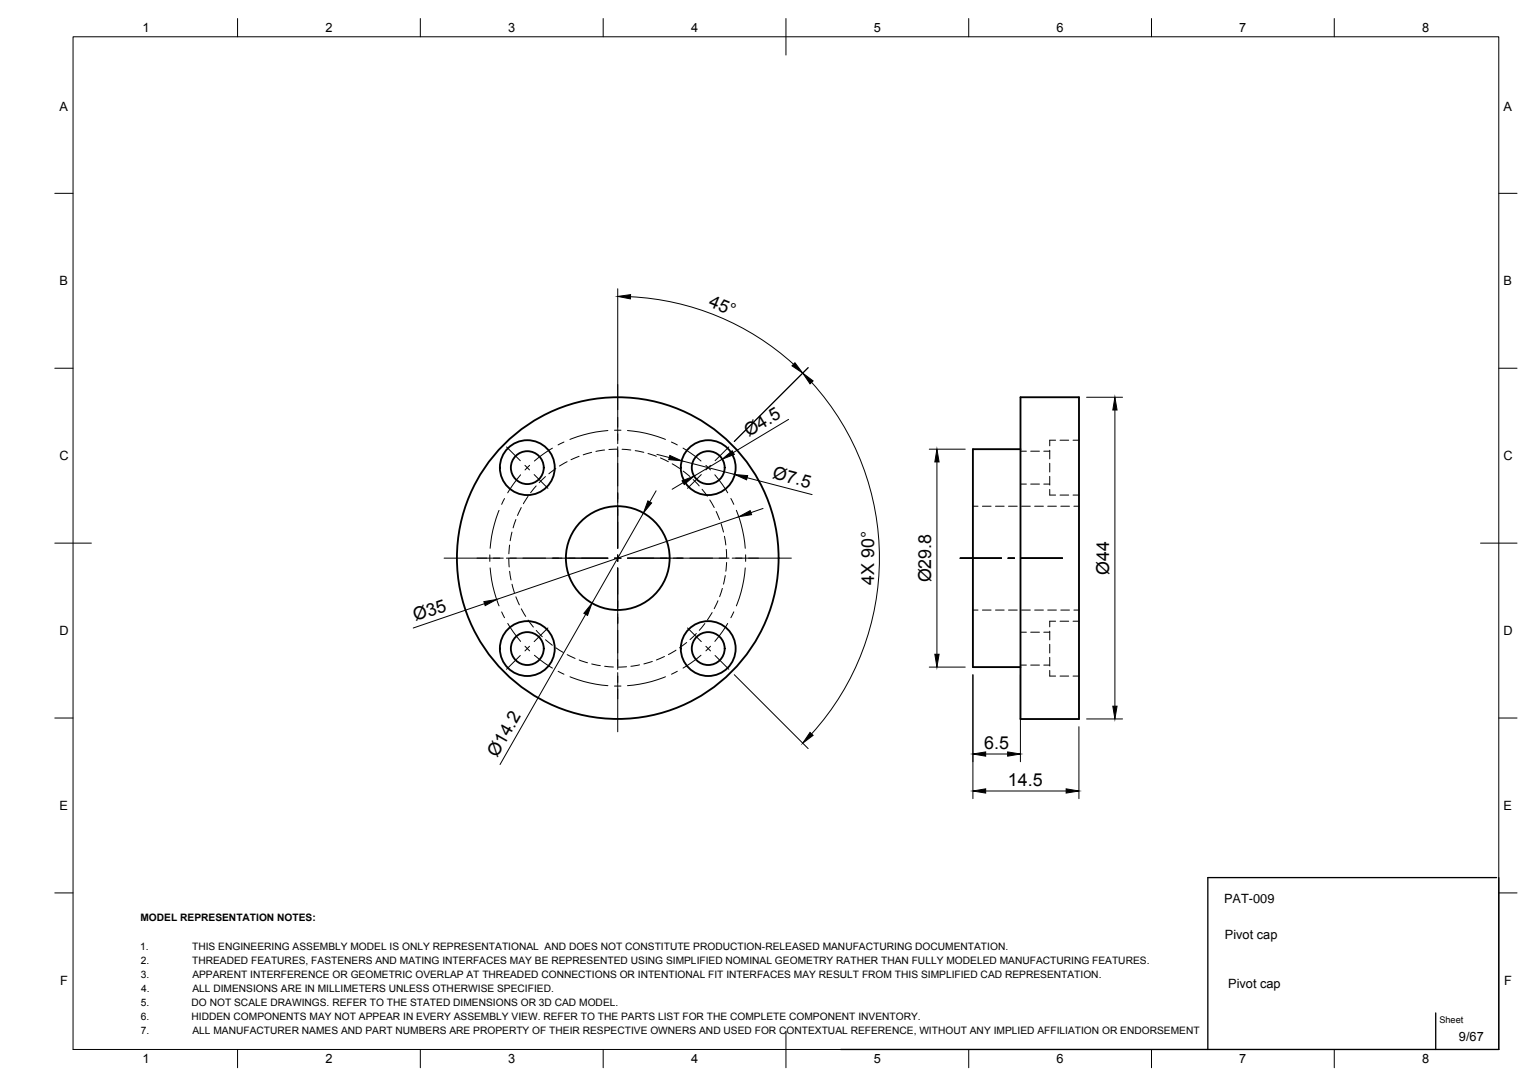
ISO-10303-21;
HEADER;
/* Generated by software containing ST-Developer
 * from STEP Tools, Inc. (www.steptools.com) 
 */

FILE_DESCRIPTION(
/* description */ ('Bell-crank linkage with push rods'),
/* implementation_level */ '2;1');

FILE_NAME(
/* name */ 'Pivot cap.step',
/* time_stamp */ '2026-10-28T03:25:15-07:00',
/* author */ (''),
/* organization */ (''),
/* preprocessor_version */ 'ST-DEVELOPER v20.2',
/* originating_system */ 'Autodesk Translation Framework v15.17.0.0',
/* authorisation */ '');

FILE_SCHEMA (('AUTOMOTIVE_DESIGN { 1 0 10303 214 3 1 1 }'));
ENDSEC;

DATA;
#10=MECHANICAL_DESIGN_GEOMETRIC_PRESENTATION_REPRESENTATION('',(#608),#16678);
#500=SHAPE_REPRESENTATION_RELATIONSHIP('SRR','None',#16916,#554);
#554=ADVANCED_BREP_SHAPE_REPRESENTATION('',(#670),#16621);
#608=STYLED_ITEM('',(#17277),#670);
#670=MANIFOLD_SOLID_BREP('Body1',#8798);
#767=FACE_BOUND('',#1872,.T.);
#768=FACE_BOUND('',#1875,.T.);
#769=FACE_BOUND('',#1878,.T.);
#770=FACE_BOUND('',#1881,.T.);
#771=FACE_BOUND('',#1888,.T.);
#772=FACE_BOUND('',#1892,.T.);
#773=FACE_BOUND('',#1893,.T.);
#774=FACE_BOUND('',#1894,.T.);
#775=FACE_BOUND('',#1895,.T.);
#776=FACE_BOUND('',#1896,.T.);
#777=FACE_BOUND('',#1898,.T.);
#778=FACE_BOUND('',#1899,.T.);
#779=FACE_BOUND('',#1900,.T.);
#780=FACE_BOUND('',#1901,.T.);
#781=FACE_BOUND('',#1902,.T.);
#996=PLANE('',#9587);
#997=PLANE('',#9592);
#998=PLANE('',#9597);
#999=PLANE('',#9602);
#1000=PLANE('',#9615);
#1001=PLANE('',#9622);
#1002=PLANE('',#9623);
#1306=FACE_OUTER_BOUND('',#1870,.T.);
#1307=FACE_OUTER_BOUND('',#1871,.T.);
#1308=FACE_OUTER_BOUND('',#1873,.T.);
#1309=FACE_OUTER_BOUND('',#1874,.T.);
#1310=FACE_OUTER_BOUND('',#1876,.T.);
#1311=FACE_OUTER_BOUND('',#1877,.T.);
#1312=FACE_OUTER_BOUND('',#1879,.T.);
#1313=FACE_OUTER_BOUND('',#1880,.T.);
#1314=FACE_OUTER_BOUND('',#1882,.T.);
#1315=FACE_OUTER_BOUND('',#1883,.T.);
#1316=FACE_OUTER_BOUND('',#1884,.T.);
#1317=FACE_OUTER_BOUND('',#1885,.T.);
#1318=FACE_OUTER_BOUND('',#1886,.T.);
#1319=FACE_OUTER_BOUND('',#1887,.T.);
#1320=FACE_OUTER_BOUND('',#1889,.T.);
#1321=FACE_OUTER_BOUND('',#1890,.T.);
#1322=FACE_OUTER_BOUND('',#1891,.T.);
#1323=FACE_OUTER_BOUND('',#1897,.T.);
#1870=EDGE_LOOP('',(#6185,#6186,#6187,#6188));
#1871=EDGE_LOOP('',(#6189));
#1872=EDGE_LOOP('',(#6190));
#1873=EDGE_LOOP('',(#6191,#6192,#6193,#6194));
#1874=EDGE_LOOP('',(#6195));
#1875=EDGE_LOOP('',(#6196));
#1876=EDGE_LOOP('',(#6197,#6198,#6199,#6200));
#1877=EDGE_LOOP('',(#6201));
#1878=EDGE_LOOP('',(#6202));
#1879=EDGE_LOOP('',(#6203,#6204,#6205,#6206));
#1880=EDGE_LOOP('',(#6207));
#1881=EDGE_LOOP('',(#6208));
#1882=EDGE_LOOP('',(#6209,#6210,#6211,#6212));
#1883=EDGE_LOOP('',(#6213,#6214,#6215,#6216));
#1884=EDGE_LOOP('',(#6217,#6218,#6219,#6220));
#1885=EDGE_LOOP('',(#6221,#6222,#6223,#6224));
#1886=EDGE_LOOP('',(#6225,#6226,#6227,#6228));
#1887=EDGE_LOOP('',(#6229));
#1888=EDGE_LOOP('',(#6230));
#1889=EDGE_LOOP('',(#6231,#6232,#6233,#6234));
#1890=EDGE_LOOP('',(#6235,#6236,#6237,#6238));
#1891=EDGE_LOOP('',(#6239));
#1892=EDGE_LOOP('',(#6240));
#1893=EDGE_LOOP('',(#6241));
#1894=EDGE_LOOP('',(#6242));
#1895=EDGE_LOOP('',(#6243));
#1896=EDGE_LOOP('',(#6244));
#1897=EDGE_LOOP('',(#6245));
#1898=EDGE_LOOP('',(#6246));
#1899=EDGE_LOOP('',(#6247));
#1900=EDGE_LOOP('',(#6248));
#1901=EDGE_LOOP('',(#6249));
#1902=EDGE_LOOP('',(#6250));
#2601=LINE('',#13898,#3150);
#2602=LINE('',#13907,#3151);
#2603=LINE('',#13916,#3152);
#2604=LINE('',#13925,#3153);
#2605=LINE('',#13933,#3154);
#2606=LINE('',#13937,#3155);
#2607=LINE('',#13941,#3156);
#2608=LINE('',#13945,#3157);
#2609=LINE('',#13950,#3158);
#2610=LINE('',#13958,#3159);
#2611=LINE('',#13963,#3160);
#3150=VECTOR('',#10963,0.375);
#3151=VECTOR('',#10974,0.375);
#3152=VECTOR('',#10985,0.375);
#3153=VECTOR('',#10996,0.375);
#3154=VECTOR('',#11007,0.225);
#3155=VECTOR('',#11012,0.225);
#3156=VECTOR('',#11017,0.225);
#3157=VECTOR('',#11022,0.225);
#3158=VECTOR('',#11027,1.49);
#3159=VECTOR('',#11038,0.71);
#3160=VECTOR('',#11043,2.2);
#3694=CIRCLE('',#9585,0.375);
#3695=CIRCLE('',#9586,0.375);
#3696=CIRCLE('',#9588,0.225);
#3697=CIRCLE('',#9590,0.375);
#3698=CIRCLE('',#9591,0.375);
#3699=CIRCLE('',#9593,0.225);
#3700=CIRCLE('',#9595,0.375);
#3701=CIRCLE('',#9596,0.375);
#3702=CIRCLE('',#9598,0.225);
#3703=CIRCLE('',#9600,0.375);
#3704=CIRCLE('',#9601,0.375);
#3705=CIRCLE('',#9603,0.225);
#3706=CIRCLE('',#9605,0.225);
#3707=CIRCLE('',#9607,0.225);
#3708=CIRCLE('',#9609,0.225);
#3709=CIRCLE('',#9611,0.225);
#3710=CIRCLE('',#9613,1.49);
#3711=CIRCLE('',#9614,1.49);
#3712=CIRCLE('',#9616,0.71);
#3713=CIRCLE('',#9618,0.71);
#3714=CIRCLE('',#9620,2.2);
#3715=CIRCLE('',#9621,2.2);
#4212=VERTEX_POINT('',#13895);
#4213=VERTEX_POINT('',#13897);
#4214=VERTEX_POINT('',#13901);
#4215=VERTEX_POINT('',#13904);
#4216=VERTEX_POINT('',#13906);
#4217=VERTEX_POINT('',#13910);
#4218=VERTEX_POINT('',#13913);
#4219=VERTEX_POINT('',#13915);
#4220=VERTEX_POINT('',#13919);
#4221=VERTEX_POINT('',#13922);
#4222=VERTEX_POINT('',#13924);
#4223=VERTEX_POINT('',#13928);
#4224=VERTEX_POINT('',#13931);
#4225=VERTEX_POINT('',#13935);
#4226=VERTEX_POINT('',#13939);
#4227=VERTEX_POINT('',#13943);
#4228=VERTEX_POINT('',#13947);
#4229=VERTEX_POINT('',#13949);
#4230=VERTEX_POINT('',#13953);
#4231=VERTEX_POINT('',#13956);
#4232=VERTEX_POINT('',#13960);
#4233=VERTEX_POINT('',#13962);
#4970=EDGE_CURVE('',#4212,#4212,#3694,.T.);
#4971=EDGE_CURVE('',#4212,#4213,#2601,.T.);
#4972=EDGE_CURVE('',#4213,#4213,#3695,.T.);
#4973=EDGE_CURVE('',#4214,#4214,#3696,.T.);
#4974=EDGE_CURVE('',#4215,#4215,#3697,.T.);
#4975=EDGE_CURVE('',#4215,#4216,#2602,.T.);
#4976=EDGE_CURVE('',#4216,#4216,#3698,.T.);
#4977=EDGE_CURVE('',#4217,#4217,#3699,.T.);
#4978=EDGE_CURVE('',#4218,#4218,#3700,.T.);
#4979=EDGE_CURVE('',#4218,#4219,#2603,.T.);
#4980=EDGE_CURVE('',#4219,#4219,#3701,.T.);
#4981=EDGE_CURVE('',#4220,#4220,#3702,.T.);
#4982=EDGE_CURVE('',#4221,#4221,#3703,.T.);
#4983=EDGE_CURVE('',#4221,#4222,#2604,.T.);
#4984=EDGE_CURVE('',#4222,#4222,#3704,.T.);
#4985=EDGE_CURVE('',#4223,#4223,#3705,.T.);
#4986=EDGE_CURVE('',#4224,#4224,#3706,.T.);
#4987=EDGE_CURVE('',#4224,#4214,#2605,.T.);
#4988=EDGE_CURVE('',#4225,#4225,#3707,.T.);
#4989=EDGE_CURVE('',#4225,#4217,#2606,.T.);
#4990=EDGE_CURVE('',#4226,#4226,#3708,.T.);
#4991=EDGE_CURVE('',#4226,#4220,#2607,.T.);
#4992=EDGE_CURVE('',#4227,#4227,#3709,.T.);
#4993=EDGE_CURVE('',#4227,#4223,#2608,.T.);
#4994=EDGE_CURVE('',#4228,#4228,#3710,.T.);
#4995=EDGE_CURVE('',#4228,#4229,#2609,.T.);
#4996=EDGE_CURVE('',#4229,#4229,#3711,.T.);
#4997=EDGE_CURVE('',#4230,#4230,#3712,.T.);
#4998=EDGE_CURVE('',#4231,#4231,#3713,.T.);
#4999=EDGE_CURVE('',#4231,#4230,#2610,.T.);
#5000=EDGE_CURVE('',#4232,#4232,#3714,.T.);
#5001=EDGE_CURVE('',#4232,#4233,#2611,.T.);
#5002=EDGE_CURVE('',#4233,#4233,#3715,.T.);
#6185=ORIENTED_EDGE('',*,*,#4970,.F.);
#6186=ORIENTED_EDGE('',*,*,#4971,.T.);
#6187=ORIENTED_EDGE('',*,*,#4972,.F.);
#6188=ORIENTED_EDGE('',*,*,#4971,.F.);
#6189=ORIENTED_EDGE('',*,*,#4970,.T.);
#6190=ORIENTED_EDGE('',*,*,#4973,.F.);
#6191=ORIENTED_EDGE('',*,*,#4974,.F.);
#6192=ORIENTED_EDGE('',*,*,#4975,.T.);
#6193=ORIENTED_EDGE('',*,*,#4976,.F.);
#6194=ORIENTED_EDGE('',*,*,#4975,.F.);
#6195=ORIENTED_EDGE('',*,*,#4974,.T.);
#6196=ORIENTED_EDGE('',*,*,#4977,.F.);
#6197=ORIENTED_EDGE('',*,*,#4978,.F.);
#6198=ORIENTED_EDGE('',*,*,#4979,.T.);
#6199=ORIENTED_EDGE('',*,*,#4980,.F.);
#6200=ORIENTED_EDGE('',*,*,#4979,.F.);
#6201=ORIENTED_EDGE('',*,*,#4978,.T.);
#6202=ORIENTED_EDGE('',*,*,#4981,.F.);
#6203=ORIENTED_EDGE('',*,*,#4982,.F.);
#6204=ORIENTED_EDGE('',*,*,#4983,.T.);
#6205=ORIENTED_EDGE('',*,*,#4984,.F.);
#6206=ORIENTED_EDGE('',*,*,#4983,.F.);
#6207=ORIENTED_EDGE('',*,*,#4982,.T.);
#6208=ORIENTED_EDGE('',*,*,#4985,.F.);
#6209=ORIENTED_EDGE('',*,*,#4986,.F.);
#6210=ORIENTED_EDGE('',*,*,#4987,.T.);
#6211=ORIENTED_EDGE('',*,*,#4973,.T.);
#6212=ORIENTED_EDGE('',*,*,#4987,.F.);
#6213=ORIENTED_EDGE('',*,*,#4988,.F.);
#6214=ORIENTED_EDGE('',*,*,#4989,.T.);
#6215=ORIENTED_EDGE('',*,*,#4977,.T.);
#6216=ORIENTED_EDGE('',*,*,#4989,.F.);
#6217=ORIENTED_EDGE('',*,*,#4990,.F.);
#6218=ORIENTED_EDGE('',*,*,#4991,.T.);
#6219=ORIENTED_EDGE('',*,*,#4981,.T.);
#6220=ORIENTED_EDGE('',*,*,#4991,.F.);
#6221=ORIENTED_EDGE('',*,*,#4992,.F.);
#6222=ORIENTED_EDGE('',*,*,#4993,.T.);
#6223=ORIENTED_EDGE('',*,*,#4985,.T.);
#6224=ORIENTED_EDGE('',*,*,#4993,.F.);
#6225=ORIENTED_EDGE('',*,*,#4994,.F.);
#6226=ORIENTED_EDGE('',*,*,#4995,.T.);
#6227=ORIENTED_EDGE('',*,*,#4996,.T.);
#6228=ORIENTED_EDGE('',*,*,#4995,.F.);
#6229=ORIENTED_EDGE('',*,*,#4996,.F.);
#6230=ORIENTED_EDGE('',*,*,#4997,.F.);
#6231=ORIENTED_EDGE('',*,*,#4998,.F.);
#6232=ORIENTED_EDGE('',*,*,#4999,.T.);
#6233=ORIENTED_EDGE('',*,*,#4997,.T.);
#6234=ORIENTED_EDGE('',*,*,#4999,.F.);
#6235=ORIENTED_EDGE('',*,*,#5000,.F.);
#6236=ORIENTED_EDGE('',*,*,#5001,.T.);
#6237=ORIENTED_EDGE('',*,*,#5002,.T.);
#6238=ORIENTED_EDGE('',*,*,#5001,.F.);
#6239=ORIENTED_EDGE('',*,*,#5000,.T.);
#6240=ORIENTED_EDGE('',*,*,#4998,.T.);
#6241=ORIENTED_EDGE('',*,*,#4984,.T.);
#6242=ORIENTED_EDGE('',*,*,#4980,.T.);
#6243=ORIENTED_EDGE('',*,*,#4976,.T.);
#6244=ORIENTED_EDGE('',*,*,#4972,.T.);
#6245=ORIENTED_EDGE('',*,*,#5002,.F.);
#6246=ORIENTED_EDGE('',*,*,#4994,.T.);
#6247=ORIENTED_EDGE('',*,*,#4992,.T.);
#6248=ORIENTED_EDGE('',*,*,#4990,.T.);
#6249=ORIENTED_EDGE('',*,*,#4988,.T.);
#6250=ORIENTED_EDGE('',*,*,#4986,.T.);
#8096=CYLINDRICAL_SURFACE('',#9584,0.375);
#8097=CYLINDRICAL_SURFACE('',#9589,0.375);
#8098=CYLINDRICAL_SURFACE('',#9594,0.375);
#8099=CYLINDRICAL_SURFACE('',#9599,0.375);
#8100=CYLINDRICAL_SURFACE('',#9604,0.225);
#8101=CYLINDRICAL_SURFACE('',#9606,0.225);
#8102=CYLINDRICAL_SURFACE('',#9608,0.225);
#8103=CYLINDRICAL_SURFACE('',#9610,0.225);
#8104=CYLINDRICAL_SURFACE('',#9612,1.49);
#8105=CYLINDRICAL_SURFACE('',#9617,0.71);
#8106=CYLINDRICAL_SURFACE('',#9619,2.2);
#8331=ADVANCED_FACE('',(#1306),#8096,.F.);
#8332=ADVANCED_FACE('',(#1307,#767),#996,.T.);
#8333=ADVANCED_FACE('',(#1308),#8097,.F.);
#8334=ADVANCED_FACE('',(#1309,#768),#997,.T.);
#8335=ADVANCED_FACE('',(#1310),#8098,.F.);
#8336=ADVANCED_FACE('',(#1311,#769),#998,.T.);
#8337=ADVANCED_FACE('',(#1312),#8099,.F.);
#8338=ADVANCED_FACE('',(#1313,#770),#999,.T.);
#8339=ADVANCED_FACE('',(#1314),#8100,.F.);
#8340=ADVANCED_FACE('',(#1315),#8101,.F.);
#8341=ADVANCED_FACE('',(#1316),#8102,.F.);
#8342=ADVANCED_FACE('',(#1317),#8103,.F.);
#8343=ADVANCED_FACE('',(#1318),#8104,.T.);
#8344=ADVANCED_FACE('',(#1319,#771),#1000,.F.);
#8345=ADVANCED_FACE('',(#1320),#8105,.F.);
#8346=ADVANCED_FACE('',(#1321),#8106,.T.);
#8347=ADVANCED_FACE('',(#1322,#772,#773,#774,#775,#776),#1001,.T.);
#8348=ADVANCED_FACE('',(#1323,#777,#778,#779,#780,#781),#1002,.F.);
#8798=CLOSED_SHELL('',(#8331,#8332,#8333,#8334,#8335,#8336,#8337,#8338,
#8339,#8340,#8341,#8342,#8343,#8344,#8345,#8346,#8347,#8348));
#9583=AXIS2_PLACEMENT_3D('',#13893,#10957,#10958);
#9584=AXIS2_PLACEMENT_3D('',#13894,#10959,#10960);
#9585=AXIS2_PLACEMENT_3D('',#13896,#10961,#10962);
#9586=AXIS2_PLACEMENT_3D('',#13899,#10964,#10965);
#9587=AXIS2_PLACEMENT_3D('',#13900,#10966,#10967);
#9588=AXIS2_PLACEMENT_3D('',#13902,#10968,#10969);
#9589=AXIS2_PLACEMENT_3D('',#13903,#10970,#10971);
#9590=AXIS2_PLACEMENT_3D('',#13905,#10972,#10973);
#9591=AXIS2_PLACEMENT_3D('',#13908,#10975,#10976);
#9592=AXIS2_PLACEMENT_3D('',#13909,#10977,#10978);
#9593=AXIS2_PLACEMENT_3D('',#13911,#10979,#10980);
#9594=AXIS2_PLACEMENT_3D('',#13912,#10981,#10982);
#9595=AXIS2_PLACEMENT_3D('',#13914,#10983,#10984);
#9596=AXIS2_PLACEMENT_3D('',#13917,#10986,#10987);
#9597=AXIS2_PLACEMENT_3D('',#13918,#10988,#10989);
#9598=AXIS2_PLACEMENT_3D('',#13920,#10990,#10991);
#9599=AXIS2_PLACEMENT_3D('',#13921,#10992,#10993);
#9600=AXIS2_PLACEMENT_3D('',#13923,#10994,#10995);
#9601=AXIS2_PLACEMENT_3D('',#13926,#10997,#10998);
#9602=AXIS2_PLACEMENT_3D('',#13927,#10999,#11000);
#9603=AXIS2_PLACEMENT_3D('',#13929,#11001,#11002);
#9604=AXIS2_PLACEMENT_3D('',#13930,#11003,#11004);
#9605=AXIS2_PLACEMENT_3D('',#13932,#11005,#11006);
#9606=AXIS2_PLACEMENT_3D('',#13934,#11008,#11009);
#9607=AXIS2_PLACEMENT_3D('',#13936,#11010,#11011);
#9608=AXIS2_PLACEMENT_3D('',#13938,#11013,#11014);
#9609=AXIS2_PLACEMENT_3D('',#13940,#11015,#11016);
#9610=AXIS2_PLACEMENT_3D('',#13942,#11018,#11019);
#9611=AXIS2_PLACEMENT_3D('',#13944,#11020,#11021);
#9612=AXIS2_PLACEMENT_3D('',#13946,#11023,#11024);
#9613=AXIS2_PLACEMENT_3D('',#13948,#11025,#11026);
#9614=AXIS2_PLACEMENT_3D('',#13951,#11028,#11029);
#9615=AXIS2_PLACEMENT_3D('',#13952,#11030,#11031);
#9616=AXIS2_PLACEMENT_3D('',#13954,#11032,#11033);
#9617=AXIS2_PLACEMENT_3D('',#13955,#11034,#11035);
#9618=AXIS2_PLACEMENT_3D('',#13957,#11036,#11037);
#9619=AXIS2_PLACEMENT_3D('',#13959,#11039,#11040);
#9620=AXIS2_PLACEMENT_3D('',#13961,#11041,#11042);
#9621=AXIS2_PLACEMENT_3D('',#13964,#11044,#11045);
#9622=AXIS2_PLACEMENT_3D('',#13965,#11046,#11047);
#9623=AXIS2_PLACEMENT_3D('',#13966,#11048,#11049);
#10957=DIRECTION('axis',(0.,0.,1.));
#10958=DIRECTION('refdir',(1.,0.,0.));
#10959=DIRECTION('center_axis',(0.,0.,1.));
#10960=DIRECTION('ref_axis',(1.,0.,0.));
#10961=DIRECTION('center_axis',(0.,0.,1.));
#10962=DIRECTION('ref_axis',(1.,0.,0.));
#10963=DIRECTION('',(0.,0.,1.));
#10964=DIRECTION('center_axis',(0.,0.,-1.));
#10965=DIRECTION('ref_axis',(1.,0.,0.));
#10966=DIRECTION('center_axis',(0.,0.,1.));
#10967=DIRECTION('ref_axis',(1.,0.,0.));
#10968=DIRECTION('center_axis',(0.,0.,1.));
#10969=DIRECTION('ref_axis',(1.,0.,0.));
#10970=DIRECTION('center_axis',(0.,0.,1.));
#10971=DIRECTION('ref_axis',(1.,0.,0.));
#10972=DIRECTION('center_axis',(0.,0.,1.));
#10973=DIRECTION('ref_axis',(1.,0.,0.));
#10974=DIRECTION('',(0.,0.,1.));
#10975=DIRECTION('center_axis',(0.,0.,-1.));
#10976=DIRECTION('ref_axis',(1.,0.,0.));
#10977=DIRECTION('center_axis',(0.,0.,1.));
#10978=DIRECTION('ref_axis',(1.,0.,0.));
#10979=DIRECTION('center_axis',(0.,0.,1.));
#10980=DIRECTION('ref_axis',(1.,0.,0.));
#10981=DIRECTION('center_axis',(0.,0.,1.));
#10982=DIRECTION('ref_axis',(1.,0.,0.));
#10983=DIRECTION('center_axis',(0.,0.,1.));
#10984=DIRECTION('ref_axis',(1.,0.,0.));
#10985=DIRECTION('',(0.,0.,1.));
#10986=DIRECTION('center_axis',(0.,0.,-1.));
#10987=DIRECTION('ref_axis',(1.,0.,0.));
#10988=DIRECTION('center_axis',(0.,0.,1.));
#10989=DIRECTION('ref_axis',(1.,0.,0.));
#10990=DIRECTION('center_axis',(0.,0.,1.));
#10991=DIRECTION('ref_axis',(1.,0.,0.));
#10992=DIRECTION('center_axis',(0.,0.,1.));
#10993=DIRECTION('ref_axis',(1.,0.,0.));
#10994=DIRECTION('center_axis',(0.,0.,1.));
#10995=DIRECTION('ref_axis',(1.,0.,0.));
#10996=DIRECTION('',(0.,0.,1.));
#10997=DIRECTION('center_axis',(0.,0.,-1.));
#10998=DIRECTION('ref_axis',(1.,0.,0.));
#10999=DIRECTION('center_axis',(0.,0.,1.));
#11000=DIRECTION('ref_axis',(1.,0.,0.));
#11001=DIRECTION('center_axis',(0.,0.,1.));
#11002=DIRECTION('ref_axis',(1.,0.,0.));
#11003=DIRECTION('center_axis',(0.,0.,1.));
#11004=DIRECTION('ref_axis',(1.,0.,0.));
#11005=DIRECTION('center_axis',(0.,0.,1.));
#11006=DIRECTION('ref_axis',(1.,0.,0.));
#11007=DIRECTION('',(0.,0.,1.));
#11008=DIRECTION('center_axis',(0.,0.,1.));
#11009=DIRECTION('ref_axis',(1.,0.,0.));
#11010=DIRECTION('center_axis',(0.,0.,1.));
#11011=DIRECTION('ref_axis',(1.,0.,0.));
#11012=DIRECTION('',(0.,0.,1.));
#11013=DIRECTION('center_axis',(0.,0.,1.));
#11014=DIRECTION('ref_axis',(1.,0.,0.));
#11015=DIRECTION('center_axis',(0.,0.,1.));
#11016=DIRECTION('ref_axis',(1.,0.,0.));
#11017=DIRECTION('',(0.,0.,1.));
#11018=DIRECTION('center_axis',(0.,0.,1.));
#11019=DIRECTION('ref_axis',(1.,0.,0.));
#11020=DIRECTION('center_axis',(0.,0.,1.));
#11021=DIRECTION('ref_axis',(1.,0.,0.));
#11022=DIRECTION('',(0.,0.,1.));
#11023=DIRECTION('center_axis',(0.,0.,1.));
#11024=DIRECTION('ref_axis',(1.,0.,0.));
#11025=DIRECTION('center_axis',(0.,0.,1.));
#11026=DIRECTION('ref_axis',(1.,0.,0.));
#11027=DIRECTION('',(0.,0.,-1.));
#11028=DIRECTION('center_axis',(0.,0.,1.));
#11029=DIRECTION('ref_axis',(1.,0.,0.));
#11030=DIRECTION('center_axis',(0.,0.,1.));
#11031=DIRECTION('ref_axis',(1.,0.,0.));
#11032=DIRECTION('center_axis',(0.,0.,-1.));
#11033=DIRECTION('ref_axis',(1.,0.,0.));
#11034=DIRECTION('center_axis',(0.,0.,1.));
#11035=DIRECTION('ref_axis',(1.,0.,0.));
#11036=DIRECTION('center_axis',(0.,0.,-1.));
#11037=DIRECTION('ref_axis',(1.,0.,0.));
#11038=DIRECTION('',(0.,0.,-1.));
#11039=DIRECTION('center_axis',(0.,0.,1.));
#11040=DIRECTION('ref_axis',(1.,0.,0.));
#11041=DIRECTION('center_axis',(0.,0.,1.));
#11042=DIRECTION('ref_axis',(1.,0.,0.));
#11043=DIRECTION('',(0.,0.,-1.));
#11044=DIRECTION('center_axis',(0.,0.,1.));
#11045=DIRECTION('ref_axis',(1.,0.,0.));
#11046=DIRECTION('center_axis',(0.,0.,1.));
#11047=DIRECTION('ref_axis',(1.,0.,0.));
#11048=DIRECTION('center_axis',(0.,0.,1.));
#11049=DIRECTION('ref_axis',(1.,0.,0.));
#13893=CARTESIAN_POINT('',(0.,0.,0.));
#13894=CARTESIAN_POINT('Origin',(-1.23743686707646,-1.23743686707646,4.));
#13895=CARTESIAN_POINT('',(-1.61243686707646,-1.23743686707646,4.));
#13896=CARTESIAN_POINT('Origin',(-1.23743686707646,-1.23743686707646,4.));
#13897=CARTESIAN_POINT('',(-1.61243686707646,-1.23743686707646,4.4));
#13898=CARTESIAN_POINT('',(-1.61243686707646,-1.23743686707646,4.));
#13899=CARTESIAN_POINT('Origin',(-1.23743686707646,-1.23743686707646,4.4));
#13900=CARTESIAN_POINT('Origin',(-1.23743686707646,-1.23743686707646,4.));
#13901=CARTESIAN_POINT('',(-1.46243686707646,-1.23743686707646,4.));
#13902=CARTESIAN_POINT('Origin',(-1.23743686707646,-1.23743686707646,4.));
#13903=CARTESIAN_POINT('Origin',(-1.23743686707646,1.23743686707646,4.));
#13904=CARTESIAN_POINT('',(-1.61243686707646,1.23743686707646,4.));
#13905=CARTESIAN_POINT('Origin',(-1.23743686707646,1.23743686707646,4.));
#13906=CARTESIAN_POINT('',(-1.61243686707646,1.23743686707646,4.4));
#13907=CARTESIAN_POINT('',(-1.61243686707646,1.23743686707646,4.));
#13908=CARTESIAN_POINT('Origin',(-1.23743686707646,1.23743686707646,4.4));
#13909=CARTESIAN_POINT('Origin',(-1.23743686707646,1.23743686707646,4.));
#13910=CARTESIAN_POINT('',(-1.46243686707646,1.23743686707646,4.));
#13911=CARTESIAN_POINT('Origin',(-1.23743686707646,1.23743686707646,4.));
#13912=CARTESIAN_POINT('Origin',(1.23743686707646,1.23743686707646,4.));
#13913=CARTESIAN_POINT('',(0.862436867076458,1.23743686707646,4.));
#13914=CARTESIAN_POINT('Origin',(1.23743686707646,1.23743686707646,4.));
#13915=CARTESIAN_POINT('',(0.862436867076458,1.23743686707646,4.4));
#13916=CARTESIAN_POINT('',(0.862436867076458,1.23743686707646,4.));
#13917=CARTESIAN_POINT('Origin',(1.23743686707646,1.23743686707646,4.4));
#13918=CARTESIAN_POINT('Origin',(1.23743686707646,1.23743686707646,4.));
#13919=CARTESIAN_POINT('',(1.01243686707646,1.23743686707646,4.));
#13920=CARTESIAN_POINT('Origin',(1.23743686707646,1.23743686707646,4.));
#13921=CARTESIAN_POINT('Origin',(1.23743686707646,-1.23743686707646,4.));
#13922=CARTESIAN_POINT('',(0.862436867076458,-1.23743686707646,4.));
#13923=CARTESIAN_POINT('Origin',(1.23743686707646,-1.23743686707646,4.));
#13924=CARTESIAN_POINT('',(0.862436867076458,-1.23743686707646,4.4));
#13925=CARTESIAN_POINT('',(0.862436867076458,-1.23743686707646,4.));
#13926=CARTESIAN_POINT('Origin',(1.23743686707646,-1.23743686707646,4.4));
#13927=CARTESIAN_POINT('Origin',(1.23743686707646,-1.23743686707646,4.));
#13928=CARTESIAN_POINT('',(1.01243686707646,-1.23743686707646,4.));
#13929=CARTESIAN_POINT('Origin',(1.23743686707646,-1.23743686707646,4.));
#13930=CARTESIAN_POINT('Origin',(-1.23743686707646,-1.23743686707646,3.5));
#13931=CARTESIAN_POINT('',(-1.46243686707646,-1.23743686707646,3.6));
#13932=CARTESIAN_POINT('Origin',(-1.23743686707646,-1.23743686707646,3.6));
#13933=CARTESIAN_POINT('',(-1.46243686707646,-1.23743686707646,3.5));
#13934=CARTESIAN_POINT('Origin',(-1.23743686707646,1.23743686707646,3.5));
#13935=CARTESIAN_POINT('',(-1.46243686707646,1.23743686707646,3.6));
#13936=CARTESIAN_POINT('Origin',(-1.23743686707646,1.23743686707646,3.6));
#13937=CARTESIAN_POINT('',(-1.46243686707646,1.23743686707646,3.5));
#13938=CARTESIAN_POINT('Origin',(1.23743686707646,1.23743686707646,3.5));
#13939=CARTESIAN_POINT('',(1.01243686707646,1.23743686707646,3.6));
#13940=CARTESIAN_POINT('Origin',(1.23743686707646,1.23743686707646,3.6));
#13941=CARTESIAN_POINT('',(1.01243686707646,1.23743686707646,3.5));
#13942=CARTESIAN_POINT('Origin',(1.23743686707646,-1.23743686707646,3.5));
#13943=CARTESIAN_POINT('',(1.01243686707646,-1.23743686707646,3.6));
#13944=CARTESIAN_POINT('Origin',(1.23743686707646,-1.23743686707646,3.6));
#13945=CARTESIAN_POINT('',(1.01243686707646,-1.23743686707646,3.5));
#13946=CARTESIAN_POINT('Origin',(0.,0.,2.95));
#13947=CARTESIAN_POINT('',(-1.49,-1.82472373072956E-16,3.6));
#13948=CARTESIAN_POINT('Origin',(0.,0.,3.6));
#13949=CARTESIAN_POINT('',(-1.49,-1.82472373072956E-16,2.95));
#13950=CARTESIAN_POINT('',(-1.49,-1.82472373072956E-16,2.95));
#13951=CARTESIAN_POINT('Origin',(0.,0.,2.95));
#13952=CARTESIAN_POINT('Origin',(0.,0.,2.95));
#13953=CARTESIAN_POINT('',(-0.71,-8.69499227394621E-17,2.95));
#13954=CARTESIAN_POINT('Origin',(0.,0.,2.95));
#13955=CARTESIAN_POINT('Origin',(0.,0.,3.6));
#13956=CARTESIAN_POINT('',(-0.71,-8.69499227394621E-17,4.4));
#13957=CARTESIAN_POINT('Origin',(0.,0.,4.4));
#13958=CARTESIAN_POINT('',(-0.71,-8.69499227394621E-17,3.6));
#13959=CARTESIAN_POINT('Origin',(0.,0.,3.6));
#13960=CARTESIAN_POINT('',(-2.2,-2.69422295812418E-16,4.4));
#13961=CARTESIAN_POINT('Origin',(0.,0.,4.4));
#13962=CARTESIAN_POINT('',(-2.2,-2.69422295812418E-16,3.6));
#13963=CARTESIAN_POINT('',(-2.2,-2.69422295812418E-16,3.6));
#13964=CARTESIAN_POINT('Origin',(0.,0.,3.6));
#13965=CARTESIAN_POINT('Origin',(0.,0.,4.4));
#13966=CARTESIAN_POINT('Origin',(0.,0.,3.6));
#16557=UNCERTAINTY_MEASURE_WITH_UNIT(LENGTH_MEASURE(0.001),#16679,
'DISTANCE_ACCURACY_VALUE',
'Maximum model space distance between geometric entities at asserted c
onnectivities');
#16614=UNCERTAINTY_MEASURE_WITH_UNIT(LENGTH_MEASURE(0.001),#16679,
'DISTANCE_ACCURACY_VALUE',
'Maximum model space distance between geometric entities at asserted c
onnectivities');
#16621=(
GEOMETRIC_REPRESENTATION_CONTEXT(3)
GLOBAL_UNCERTAINTY_ASSIGNED_CONTEXT((#16557))
GLOBAL_UNIT_ASSIGNED_CONTEXT((#16679,#16681,#16682))
REPRESENTATION_CONTEXT('','3D')
);
#16678=(
GEOMETRIC_REPRESENTATION_CONTEXT(3)
GLOBAL_UNCERTAINTY_ASSIGNED_CONTEXT((#16614))
GLOBAL_UNIT_ASSIGNED_CONTEXT((#16679,#16681,#16682))
REPRESENTATION_CONTEXT('','3D')
);
#16679=(
LENGTH_UNIT()
NAMED_UNIT(*)
SI_UNIT(.CENTI.,.METRE.)
);
#16681=(
NAMED_UNIT(*)
PLANE_ANGLE_UNIT()
SI_UNIT($,.RADIAN.)
);
#16682=(
NAMED_UNIT(*)
SI_UNIT($,.STERADIAN.)
SOLID_ANGLE_UNIT()
);
#16689=SHAPE_DEFINITION_REPRESENTATION(#16752,#16916);
#16752=PRODUCT_DEFINITION_SHAPE('',$,#16980);
#16916=SHAPE_REPRESENTATION('',(#9583),#16621);
#16973=PRODUCT_DEFINITION_CONTEXT('part definition',#17164,'design');
#16980=PRODUCT_DEFINITION('Pivot cap','Pivot cap',#17043,#16973);
#17043=PRODUCT_DEFINITION_FORMATION('',$,#17172);
#17164=APPLICATION_CONTEXT(
'Core Data for Automotive Mechanical Design Process');
#17165=PRODUCT_CONTEXT('part definition',#17164,'mechanical');
#17172=PRODUCT('Pivot cap','Pivot cap','Pivot cap',(#17165));
#17271=COLOUR_RGB('Light Blue',0.38,0.62,0.78);
#17272=FILL_AREA_STYLE_COLOUR('',#17271);
#17273=FILL_AREA_STYLE('',(#17272));
#17274=SURFACE_STYLE_FILL_AREA(#17273);
#17275=SURFACE_SIDE_STYLE('',(#17274));
#17276=SURFACE_STYLE_USAGE(.BOTH.,#17275);
#17277=PRESENTATION_STYLE_ASSIGNMENT((#17276));
ENDSEC;
END-ISO-10303-21;
